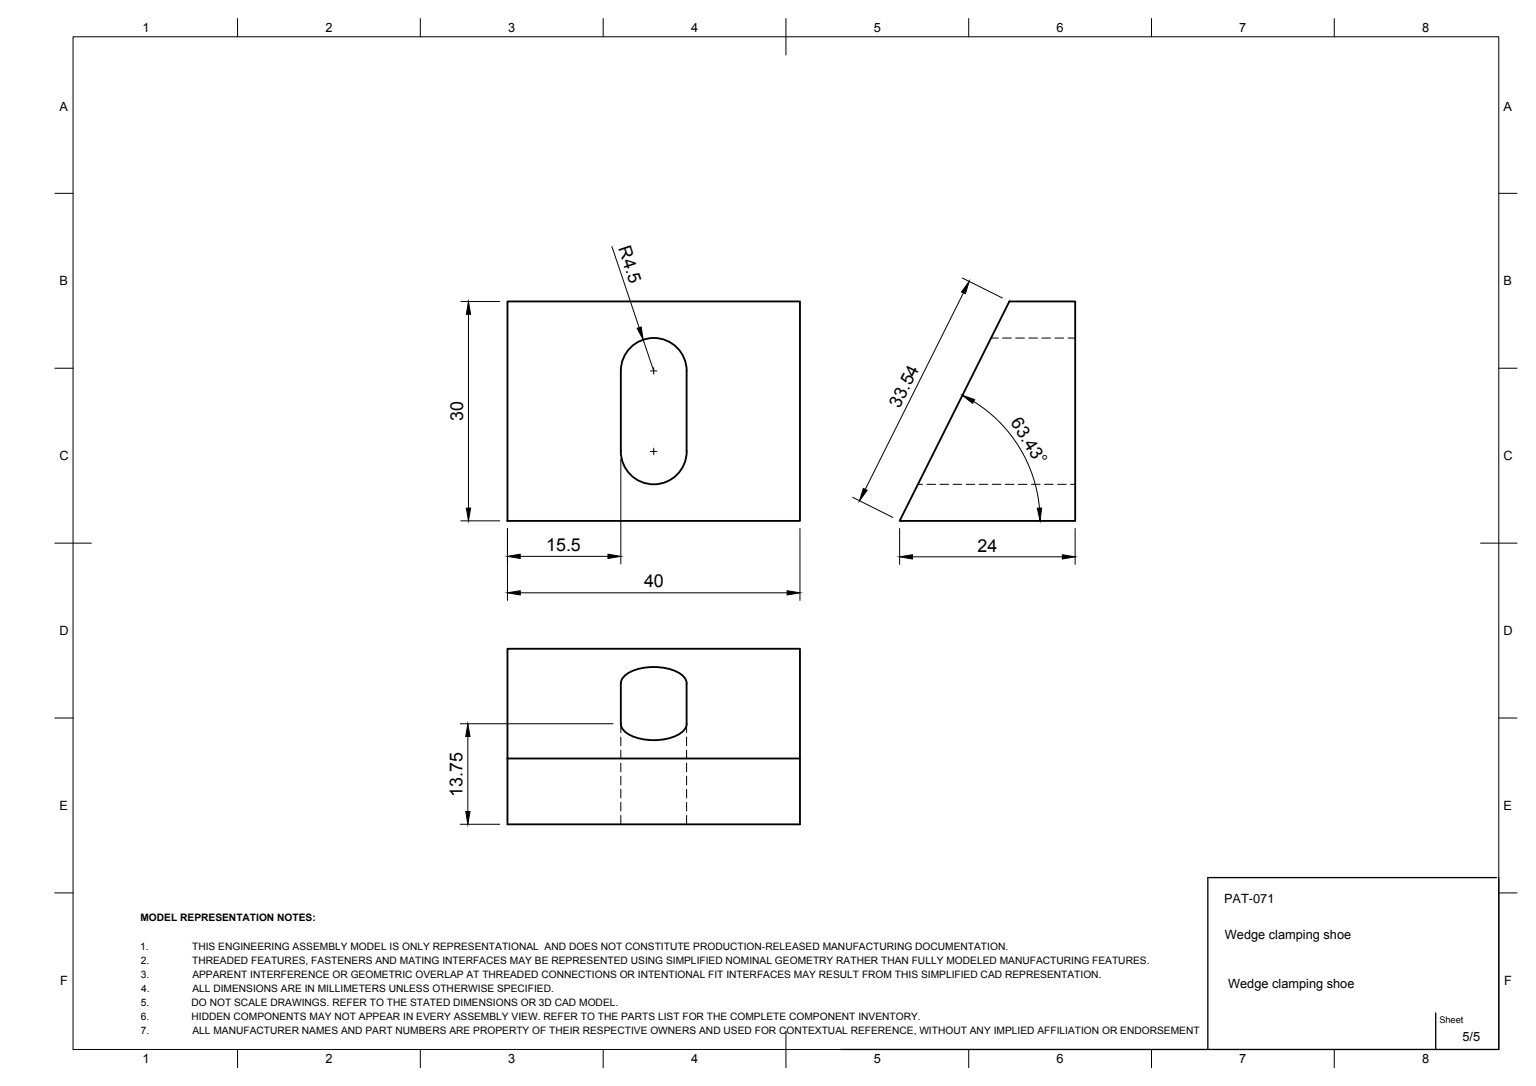
ISO-10303-21;
HEADER;
/* Generated by software containing ST-Developer
 * from STEP Tools, Inc. (www.steptools.com) 
 */

FILE_DESCRIPTION(
/* description */ ('Low-profile wedge edge clamp'),
/* implementation_level */ '2;1');

FILE_NAME(
/* name */ 'Wedge clamping shoe.step',
/* time_stamp */ '2026-10-29T15:58:13-07:00',
/* author */ (''),
/* organization */ (''),
/* preprocessor_version */ 'ST-DEVELOPER v20.2',
/* originating_system */ 'Autodesk Translation Framework v15.17.0.0',
/* authorisation */ '');

FILE_SCHEMA (('AUTOMOTIVE_DESIGN { 1 0 10303 214 3 1 1 }'));
ENDSEC;

DATA;
#10=MECHANICAL_DESIGN_GEOMETRIC_PRESENTATION_REPRESENTATION('',(#81),#2996);
#65=ELLIPSE('',#1914,0.503115294937453,0.45);
#66=ELLIPSE('',#1916,0.503115294937453,0.45);
#69=SHAPE_REPRESENTATION_RELATIONSHIP('SRR','None',#3031,#75);
#75=ADVANCED_BREP_SHAPE_REPRESENTATION('',(#87),#2992);
#81=STYLED_ITEM('',(#3140),#87);
#87=MANIFOLD_SOLID_BREP('Body1',#1710);
#156=FACE_BOUND('',#421,.T.);
#157=FACE_BOUND('',#426,.T.);
#178=PLANE('',#1908);
#179=PLANE('',#1909);
#180=PLANE('',#1910);
#181=PLANE('',#1917);
#182=PLANE('',#1918);
#183=PLANE('',#1919);
#184=PLANE('',#1920);
#185=PLANE('',#1921);
#259=FACE_OUTER_BOUND('',#418,.T.);
#260=FACE_OUTER_BOUND('',#419,.T.);
#261=FACE_OUTER_BOUND('',#420,.T.);
#262=FACE_OUTER_BOUND('',#422,.T.);
#263=FACE_OUTER_BOUND('',#423,.T.);
#264=FACE_OUTER_BOUND('',#424,.T.);
#265=FACE_OUTER_BOUND('',#425,.T.);
#266=FACE_OUTER_BOUND('',#427,.T.);
#267=FACE_OUTER_BOUND('',#428,.T.);
#268=FACE_OUTER_BOUND('',#429,.T.);
#418=EDGE_LOOP('',(#1403,#1404,#1405,#1406));
#419=EDGE_LOOP('',(#1407,#1408,#1409,#1410));
#420=EDGE_LOOP('',(#1411,#1412,#1413,#1414));
#421=EDGE_LOOP('',(#1415,#1416,#1417,#1418));
#422=EDGE_LOOP('',(#1419,#1420,#1421,#1422));
#423=EDGE_LOOP('',(#1423,#1424,#1425,#1426));
#424=EDGE_LOOP('',(#1427,#1428,#1429,#1430));
#425=EDGE_LOOP('',(#1431,#1432,#1433,#1434));
#426=EDGE_LOOP('',(#1435,#1436,#1437,#1438));
#427=EDGE_LOOP('',(#1439,#1440,#1441,#1442));
#428=EDGE_LOOP('',(#1443,#1444,#1445,#1446));
#429=EDGE_LOOP('',(#1447,#1448,#1449,#1450));
#525=LINE('',#2775,#644);
#526=LINE('',#2777,#645);
#527=LINE('',#2779,#646);
#528=LINE('',#2780,#647);
#529=LINE('',#2784,#648);
#530=LINE('',#2786,#649);
#531=LINE('',#2788,#650);
#532=LINE('',#2789,#651);
#533=LINE('',#2793,#652);
#534=LINE('',#2795,#653);
#535=LINE('',#2797,#654);
#536=LINE('',#2798,#655);
#537=LINE('',#2807,#656);
#538=LINE('',#2809,#657);
#539=LINE('',#2810,#658);
#540=LINE('',#2813,#659);
#541=LINE('',#2815,#660);
#542=LINE('',#2816,#661);
#543=LINE('',#2818,#662);
#544=LINE('',#2819,#663);
#644=VECTOR('',#2295,1.);
#645=VECTOR('',#2296,1.);
#646=VECTOR('',#2297,1.);
#647=VECTOR('',#2298,1.);
#648=VECTOR('',#2301,1.);
#649=VECTOR('',#2302,1.);
#650=VECTOR('',#2303,1.);
#651=VECTOR('',#2304,1.);
#652=VECTOR('',#2307,1.);
#653=VECTOR('',#2308,1.);
#654=VECTOR('',#2309,1.);
#655=VECTOR('',#2310,1.);
#656=VECTOR('',#2325,1.);
#657=VECTOR('',#2326,1.);
#658=VECTOR('',#2327,1.);
#659=VECTOR('',#2330,1.);
#660=VECTOR('',#2331,1.);
#661=VECTOR('',#2332,1.);
#662=VECTOR('',#2335,1.);
#663=VECTOR('',#2336,1.);
#773=CIRCLE('',#1911,0.45);
#774=CIRCLE('',#1912,0.45);
#876=VERTEX_POINT('',#2773);
#877=VERTEX_POINT('',#2774);
#878=VERTEX_POINT('',#2776);
#879=VERTEX_POINT('',#2778);
#880=VERTEX_POINT('',#2782);
#881=VERTEX_POINT('',#2783);
#882=VERTEX_POINT('',#2785);
#883=VERTEX_POINT('',#2787);
#884=VERTEX_POINT('',#2791);
#885=VERTEX_POINT('',#2792);
#886=VERTEX_POINT('',#2794);
#887=VERTEX_POINT('',#2796);
#888=VERTEX_POINT('',#2806);
#889=VERTEX_POINT('',#2808);
#890=VERTEX_POINT('',#2812);
#891=VERTEX_POINT('',#2814);
#1060=EDGE_CURVE('',#876,#877,#525,.T.);
#1061=EDGE_CURVE('',#878,#876,#526,.T.);
#1062=EDGE_CURVE('',#879,#878,#527,.T.);
#1063=EDGE_CURVE('',#879,#877,#528,.T.);
#1064=EDGE_CURVE('',#880,#881,#529,.T.);
#1065=EDGE_CURVE('',#882,#880,#530,.T.);
#1066=EDGE_CURVE('',#883,#882,#531,.T.);
#1067=EDGE_CURVE('',#881,#883,#532,.T.);
#1068=EDGE_CURVE('',#884,#885,#533,.T.);
#1069=EDGE_CURVE('',#884,#886,#534,.T.);
#1070=EDGE_CURVE('',#887,#886,#535,.T.);
#1071=EDGE_CURVE('',#885,#887,#536,.T.);
#1072=EDGE_CURVE('',#878,#883,#773,.T.);
#1073=EDGE_CURVE('',#882,#879,#774,.T.);
#1074=EDGE_CURVE('',#877,#880,#65,.T.);
#1075=EDGE_CURVE('',#881,#876,#66,.T.);
#1076=EDGE_CURVE('',#885,#888,#537,.T.);
#1077=EDGE_CURVE('',#889,#887,#538,.T.);
#1078=EDGE_CURVE('',#888,#889,#539,.T.);
#1079=EDGE_CURVE('',#888,#890,#540,.T.);
#1080=EDGE_CURVE('',#891,#889,#541,.T.);
#1081=EDGE_CURVE('',#890,#891,#542,.T.);
#1082=EDGE_CURVE('',#890,#884,#543,.T.);
#1083=EDGE_CURVE('',#886,#891,#544,.T.);
#1403=ORIENTED_EDGE('',*,*,#1060,.F.);
#1404=ORIENTED_EDGE('',*,*,#1061,.F.);
#1405=ORIENTED_EDGE('',*,*,#1062,.F.);
#1406=ORIENTED_EDGE('',*,*,#1063,.T.);
#1407=ORIENTED_EDGE('',*,*,#1064,.F.);
#1408=ORIENTED_EDGE('',*,*,#1065,.F.);
#1409=ORIENTED_EDGE('',*,*,#1066,.F.);
#1410=ORIENTED_EDGE('',*,*,#1067,.F.);
#1411=ORIENTED_EDGE('',*,*,#1068,.F.);
#1412=ORIENTED_EDGE('',*,*,#1069,.T.);
#1413=ORIENTED_EDGE('',*,*,#1070,.F.);
#1414=ORIENTED_EDGE('',*,*,#1071,.F.);
#1415=ORIENTED_EDGE('',*,*,#1062,.T.);
#1416=ORIENTED_EDGE('',*,*,#1072,.T.);
#1417=ORIENTED_EDGE('',*,*,#1066,.T.);
#1418=ORIENTED_EDGE('',*,*,#1073,.T.);
#1419=ORIENTED_EDGE('',*,*,#1063,.F.);
#1420=ORIENTED_EDGE('',*,*,#1073,.F.);
#1421=ORIENTED_EDGE('',*,*,#1065,.T.);
#1422=ORIENTED_EDGE('',*,*,#1074,.F.);
#1423=ORIENTED_EDGE('',*,*,#1061,.T.);
#1424=ORIENTED_EDGE('',*,*,#1075,.F.);
#1425=ORIENTED_EDGE('',*,*,#1067,.T.);
#1426=ORIENTED_EDGE('',*,*,#1072,.F.);
#1427=ORIENTED_EDGE('',*,*,#1076,.F.);
#1428=ORIENTED_EDGE('',*,*,#1071,.T.);
#1429=ORIENTED_EDGE('',*,*,#1077,.F.);
#1430=ORIENTED_EDGE('',*,*,#1078,.F.);
#1431=ORIENTED_EDGE('',*,*,#1079,.F.);
#1432=ORIENTED_EDGE('',*,*,#1078,.T.);
#1433=ORIENTED_EDGE('',*,*,#1080,.F.);
#1434=ORIENTED_EDGE('',*,*,#1081,.F.);
#1435=ORIENTED_EDGE('',*,*,#1060,.T.);
#1436=ORIENTED_EDGE('',*,*,#1074,.T.);
#1437=ORIENTED_EDGE('',*,*,#1064,.T.);
#1438=ORIENTED_EDGE('',*,*,#1075,.T.);
#1439=ORIENTED_EDGE('',*,*,#1082,.F.);
#1440=ORIENTED_EDGE('',*,*,#1081,.T.);
#1441=ORIENTED_EDGE('',*,*,#1083,.F.);
#1442=ORIENTED_EDGE('',*,*,#1069,.F.);
#1443=ORIENTED_EDGE('',*,*,#1070,.T.);
#1444=ORIENTED_EDGE('',*,*,#1083,.T.);
#1445=ORIENTED_EDGE('',*,*,#1080,.T.);
#1446=ORIENTED_EDGE('',*,*,#1077,.T.);
#1447=ORIENTED_EDGE('',*,*,#1068,.T.);
#1448=ORIENTED_EDGE('',*,*,#1076,.T.);
#1449=ORIENTED_EDGE('',*,*,#1079,.T.);
#1450=ORIENTED_EDGE('',*,*,#1082,.T.);
#1608=CYLINDRICAL_SURFACE('',#1913,0.45);
#1609=CYLINDRICAL_SURFACE('',#1915,0.45);
#1666=ADVANCED_FACE('',(#259),#178,.F.);
#1667=ADVANCED_FACE('',(#260),#179,.F.);
#1668=ADVANCED_FACE('',(#261,#156),#180,.T.);
#1669=ADVANCED_FACE('',(#262),#1608,.F.);
#1670=ADVANCED_FACE('',(#263),#1609,.F.);
#1671=ADVANCED_FACE('',(#264),#181,.T.);
#1672=ADVANCED_FACE('',(#265,#157),#182,.T.);
#1673=ADVANCED_FACE('',(#266),#183,.T.);
#1674=ADVANCED_FACE('',(#267),#184,.T.);
#1675=ADVANCED_FACE('',(#268),#185,.F.);
#1710=CLOSED_SHELL('',(#1666,#1667,#1668,#1669,#1670,#1671,#1672,#1673,
#1674,#1675));
#1907=AXIS2_PLACEMENT_3D('',#2771,#2291,#2292);
#1908=AXIS2_PLACEMENT_3D('',#2772,#2293,#2294);
#1909=AXIS2_PLACEMENT_3D('',#2781,#2299,#2300);
#1910=AXIS2_PLACEMENT_3D('',#2790,#2305,#2306);
#1911=AXIS2_PLACEMENT_3D('',#2799,#2311,#2312);
#1912=AXIS2_PLACEMENT_3D('',#2800,#2313,#2314);
#1913=AXIS2_PLACEMENT_3D('',#2801,#2315,#2316);
#1914=AXIS2_PLACEMENT_3D('',#2802,#2317,#2318);
#1915=AXIS2_PLACEMENT_3D('',#2803,#2319,#2320);
#1916=AXIS2_PLACEMENT_3D('',#2804,#2321,#2322);
#1917=AXIS2_PLACEMENT_3D('',#2805,#2323,#2324);
#1918=AXIS2_PLACEMENT_3D('',#2811,#2328,#2329);
#1919=AXIS2_PLACEMENT_3D('',#2817,#2333,#2334);
#1920=AXIS2_PLACEMENT_3D('',#2820,#2337,#2338);
#1921=AXIS2_PLACEMENT_3D('',#2821,#2339,#2340);
#2291=DIRECTION('axis',(0.,0.,1.));
#2292=DIRECTION('refdir',(1.,0.,0.));
#2293=DIRECTION('center_axis',(0.,1.,0.));
#2294=DIRECTION('ref_axis',(-1.,0.,0.));
#2295=DIRECTION('',(-0.894427190999916,0.,-0.447213595499958));
#2296=DIRECTION('',(0.,0.,-1.));
#2297=DIRECTION('',(1.,0.,0.));
#2298=DIRECTION('',(0.,0.,-1.));
#2299=DIRECTION('center_axis',(0.,-1.,0.));
#2300=DIRECTION('ref_axis',(1.,0.,0.));
#2301=DIRECTION('',(0.894427190999916,0.,0.447213595499958));
#2302=DIRECTION('',(0.,0.,-1.));
#2303=DIRECTION('',(-1.,0.,0.));
#2304=DIRECTION('',(0.,0.,1.));
#2305=DIRECTION('center_axis',(0.,0.,1.));
#2306=DIRECTION('ref_axis',(1.,0.,0.));
#2307=DIRECTION('',(-1.,0.,0.));
#2308=DIRECTION('',(0.,1.,0.));
#2309=DIRECTION('',(1.,0.,0.));
#2310=DIRECTION('',(0.,1.,0.));
#2311=DIRECTION('center_axis',(0.,0.,-1.));
#2312=DIRECTION('ref_axis',(1.,0.,0.));
#2313=DIRECTION('center_axis',(0.,0.,-1.));
#2314=DIRECTION('ref_axis',(1.,0.,0.));
#2315=DIRECTION('center_axis',(0.,0.,1.));
#2316=DIRECTION('ref_axis',(-1.,1.22464679914735E-16,0.));
#2317=DIRECTION('center_axis',(-0.447213595499958,0.,0.894427190999916));
#2318=DIRECTION('ref_axis',(0.894427190999916,0.,0.447213595499958));
#2319=DIRECTION('center_axis',(0.,0.,1.));
#2320=DIRECTION('ref_axis',(1.,0.,0.));
#2321=DIRECTION('center_axis',(-0.447213595499958,0.,0.894427190999916));
#2322=DIRECTION('ref_axis',(0.894427190999916,0.,0.447213595499958));
#2323=DIRECTION('center_axis',(-1.,0.,0.));
#2324=DIRECTION('ref_axis',(0.,0.,1.));
#2325=DIRECTION('',(0.,0.,-1.));
#2326=DIRECTION('',(0.,0.,1.));
#2327=DIRECTION('',(0.,1.,0.));
#2328=DIRECTION('center_axis',(0.447213595499958,0.,-0.894427190999916));
#2329=DIRECTION('ref_axis',(-0.894427190999916,0.,-0.447213595499958));
#2330=DIRECTION('',(0.894427190999916,0.,0.447213595499958));
#2331=DIRECTION('',(-0.894427190999916,0.,-0.447213595499958));
#2332=DIRECTION('',(0.,1.,0.));
#2333=DIRECTION('center_axis',(1.,0.,0.));
#2334=DIRECTION('ref_axis',(0.,0.,-1.));
#2335=DIRECTION('',(0.,0.,1.));
#2336=DIRECTION('',(0.,0.,-1.));
#2337=DIRECTION('center_axis',(0.,1.,0.));
#2338=DIRECTION('ref_axis',(0.,0.,1.));
#2339=DIRECTION('center_axis',(0.,1.,0.));
#2340=DIRECTION('ref_axis',(1.,0.,0.));
#2771=CARTESIAN_POINT('',(0.,0.,0.));
#2772=CARTESIAN_POINT('Origin',(2.05,0.45,1.5));
#2773=CARTESIAN_POINT('',(2.05,0.45,2.625));
#2774=CARTESIAN_POINT('',(0.95,0.45,2.075));
#2775=CARTESIAN_POINT('',(2.3,0.45,2.75));
#2776=CARTESIAN_POINT('',(2.05,0.45,4.));
#2777=CARTESIAN_POINT('',(2.05,0.45,1.5));
#2778=CARTESIAN_POINT('',(0.95,0.45,4.));
#2779=CARTESIAN_POINT('',(1.025,0.45,4.));
#2780=CARTESIAN_POINT('',(0.95,0.45,1.5));
#2781=CARTESIAN_POINT('Origin',(0.95,-0.45,1.5));
#2782=CARTESIAN_POINT('',(0.95,-0.45,2.075));
#2783=CARTESIAN_POINT('',(2.05,-0.45,2.625));
#2784=CARTESIAN_POINT('',(1.86,-0.45,2.53));
#2785=CARTESIAN_POINT('',(0.95,-0.45,4.));
#2786=CARTESIAN_POINT('',(0.95,-0.45,1.5));
#2787=CARTESIAN_POINT('',(2.05,-0.45,4.));
#2788=CARTESIAN_POINT('',(0.475,-0.45,4.));
#2789=CARTESIAN_POINT('',(2.05,-0.45,1.5));
#2790=CARTESIAN_POINT('Origin',(0.,-2.,4.));
#2791=CARTESIAN_POINT('',(3.,-2.,4.));
#2792=CARTESIAN_POINT('',(0.,-2.,4.));
#2793=CARTESIAN_POINT('',(3.,-2.,4.));
#2794=CARTESIAN_POINT('',(3.,2.,4.));
#2795=CARTESIAN_POINT('',(3.,-2.,4.));
#2796=CARTESIAN_POINT('',(0.,2.,4.));
#2797=CARTESIAN_POINT('',(3.,2.,4.));
#2798=CARTESIAN_POINT('',(0.,-2.,4.));
#2799=CARTESIAN_POINT('Origin',(2.05,0.,4.));
#2800=CARTESIAN_POINT('Origin',(0.95,0.,4.));
#2801=CARTESIAN_POINT('Origin',(0.95,0.,1.5));
#2802=CARTESIAN_POINT('Origin',(0.95,0.,2.075));
#2803=CARTESIAN_POINT('Origin',(2.05,0.,1.5));
#2804=CARTESIAN_POINT('Origin',(2.05,0.,2.625));
#2805=CARTESIAN_POINT('Origin',(0.,-2.,1.6));
#2806=CARTESIAN_POINT('',(0.,-2.,1.6));
#2807=CARTESIAN_POINT('',(0.,-2.,4.));
#2808=CARTESIAN_POINT('',(0.,2.,1.6));
#2809=CARTESIAN_POINT('',(0.,2.,4.));
#2810=CARTESIAN_POINT('',(0.,-2.,1.6));
#2811=CARTESIAN_POINT('Origin',(3.,-2.,3.1));
#2812=CARTESIAN_POINT('',(3.,-2.,3.1));
#2813=CARTESIAN_POINT('',(0.,-2.,1.6));
#2814=CARTESIAN_POINT('',(3.,2.,3.1));
#2815=CARTESIAN_POINT('',(0.,2.,1.6));
#2816=CARTESIAN_POINT('',(3.,-2.,3.1));
#2817=CARTESIAN_POINT('Origin',(3.,-2.,4.));
#2818=CARTESIAN_POINT('',(3.,-2.,3.1));
#2819=CARTESIAN_POINT('',(3.,2.,3.1));
#2820=CARTESIAN_POINT('Origin',(1.5,2.,2.8));
#2821=CARTESIAN_POINT('Origin',(1.5,-2.,2.8));
#2983=UNCERTAINTY_MEASURE_WITH_UNIT(LENGTH_MEASURE(0.001),#2997,
'DISTANCE_ACCURACY_VALUE',
'Maximum model space distance between geometric entities at asserted c
onnectivities');
#2987=UNCERTAINTY_MEASURE_WITH_UNIT(LENGTH_MEASURE(0.001),#2997,
'DISTANCE_ACCURACY_VALUE',
'Maximum model space distance between geometric entities at asserted c
onnectivities');
#2992=(
GEOMETRIC_REPRESENTATION_CONTEXT(3)
GLOBAL_UNCERTAINTY_ASSIGNED_CONTEXT((#2983))
GLOBAL_UNIT_ASSIGNED_CONTEXT((#2997,#2999,#3000))
REPRESENTATION_CONTEXT('','3D')
);
#2996=(
GEOMETRIC_REPRESENTATION_CONTEXT(3)
GLOBAL_UNCERTAINTY_ASSIGNED_CONTEXT((#2987))
GLOBAL_UNIT_ASSIGNED_CONTEXT((#2997,#2999,#3000))
REPRESENTATION_CONTEXT('','3D')
);
#2997=(
LENGTH_UNIT()
NAMED_UNIT(*)
SI_UNIT(.CENTI.,.METRE.)
);
#2999=(
NAMED_UNIT(*)
PLANE_ANGLE_UNIT()
SI_UNIT($,.RADIAN.)
);
#3000=(
NAMED_UNIT(*)
SI_UNIT($,.STERADIAN.)
SOLID_ANGLE_UNIT()
);
#3005=SHAPE_DEFINITION_REPRESENTATION(#3013,#3031);
#3013=PRODUCT_DEFINITION_SHAPE('',$,#3040);
#3031=SHAPE_REPRESENTATION('',(#1907),#2992);
#3035=PRODUCT_DEFINITION_CONTEXT('part definition',#3061,'design');
#3040=PRODUCT_DEFINITION('Wedge clamping shoe','Wedge clamping shoe',#3048,
#3035);
#3048=PRODUCT_DEFINITION_FORMATION('',$,#3067);
#3061=APPLICATION_CONTEXT(
'Core Data for Automotive Mechanical Design Process');
#3062=PRODUCT_CONTEXT('part definition',#3061,'mechanical');
#3067=PRODUCT('Wedge clamping shoe','Wedge clamping shoe',
'Wedge clamping shoe',(#3062));
#3134=COLOUR_RGB('Off White',0.89,0.88,0.83);
#3135=FILL_AREA_STYLE_COLOUR('',#3134);
#3136=FILL_AREA_STYLE('',(#3135));
#3137=SURFACE_STYLE_FILL_AREA(#3136);
#3138=SURFACE_SIDE_STYLE('',(#3137));
#3139=SURFACE_STYLE_USAGE(.BOTH.,#3138);
#3140=PRESENTATION_STYLE_ASSIGNMENT((#3139));
ENDSEC;
END-ISO-10303-21;
